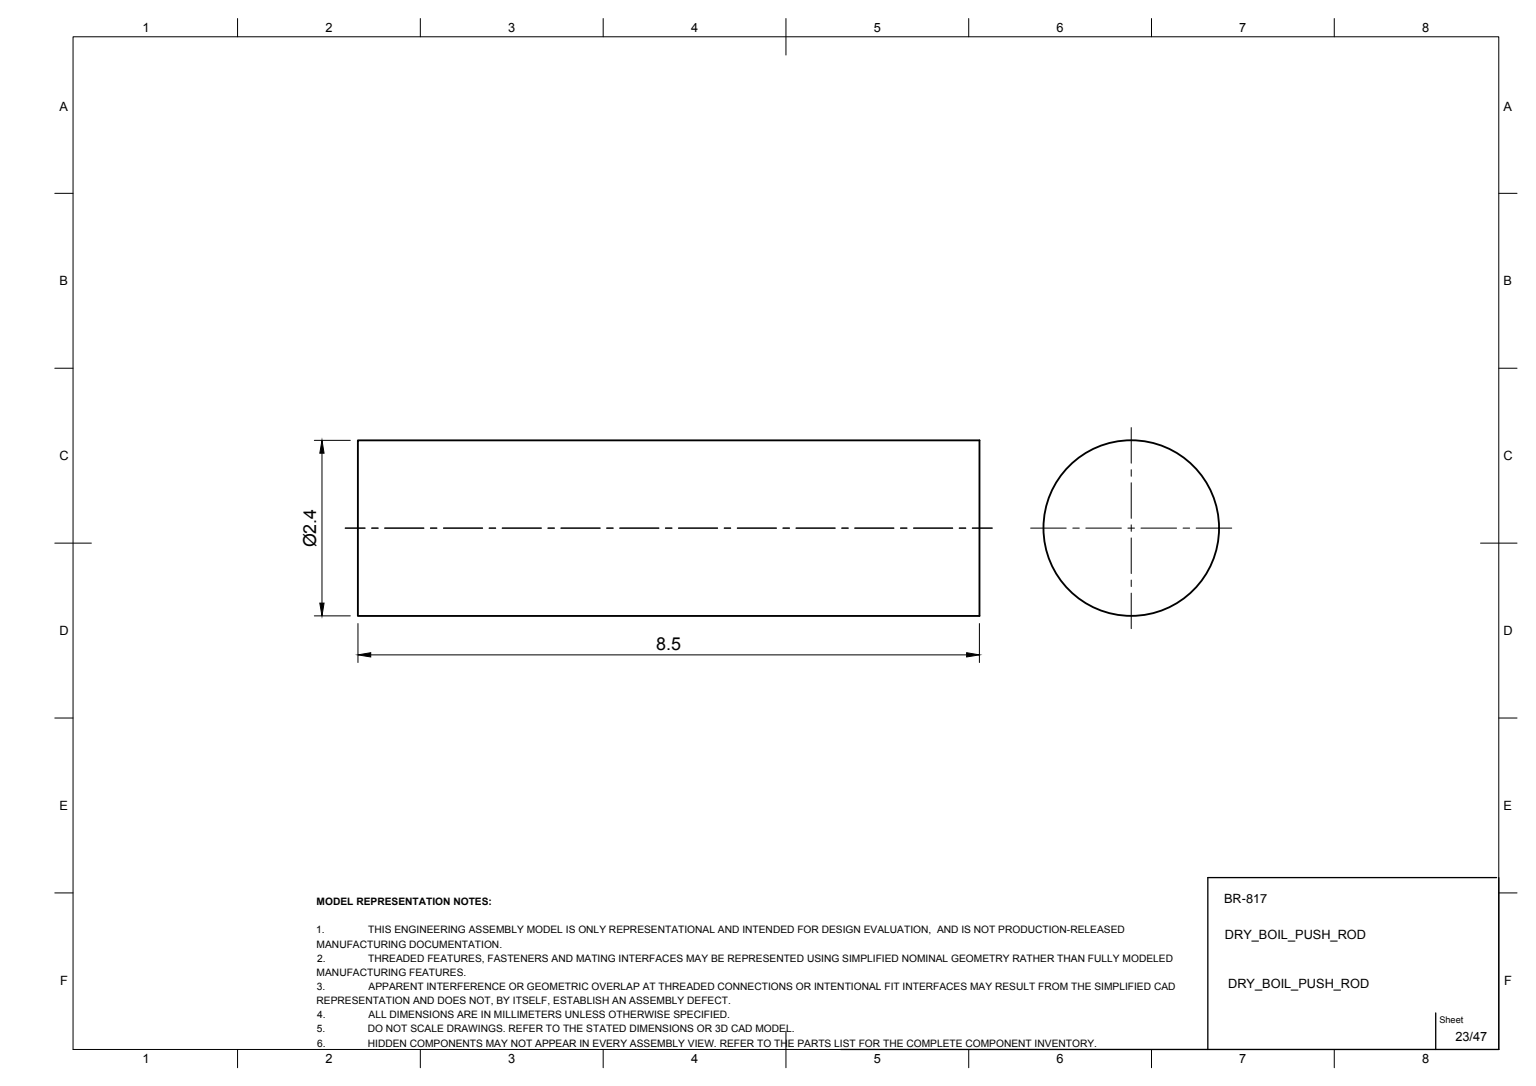
ISO-10303-21;
HEADER;
FILE_DESCRIPTION((''),'2;1');
FILE_NAME('DRY_BOIL_PUSH_ROD.step','2026-10-01T22:07:29-07:00',(''),(''),'','','');
FILE_SCHEMA (('AUTOMOTIVE_DESIGN { 1 0 10303 214 3 1 1 }'));
ENDSEC;
DATA;
#10=MECHANICAL_DESIGN_GEOMETRIC_PRESENTATION_REPRESENTATION('',(#557),#15484);
#487=SHAPE_REPRESENTATION_RELATIONSHIP('SRR','None',#15636,#522) ;
#522=ADVANCED_BREP_SHAPE_REPRESENTATION('',(#598),#15460) ;
#557=STYLED_ITEM('',(#15832),#598) ;
#598=MANIFOLD_SOLID_BREP('DRY_BOIL_PUSH_ROD',#8268) ;
#681=CYLINDRICAL_SURFACE('',#8996,0.12) ;
#1005=CIRCLE('',#8997,0.12) ;
#1006=CIRCLE('',#8998,0.12) ;
#1532=FACE_OUTER_BOUND('',#2088,.T.) ;
#1533=FACE_OUTER_BOUND('',#2089,.T.) ;
#1534=FACE_OUTER_BOUND('',#2090,.T.) ;
#2088=EDGE_LOOP('',(#5937,#5938,#5939,#5940)) ;
#2089=EDGE_LOOP('',(#5941)) ;
#2090=EDGE_LOOP('',(#5942)) ;
#2648=LINE('',#13678,#3122) ;
#3122=VECTOR('',#10765,0.12) ;
#3611=VERTEX_POINT('',#13675) ;
#3612=VERTEX_POINT('',#13677) ;
#4473=EDGE_CURVE('',#3611,#3611,#1005,.T.) ;
#4474=EDGE_CURVE('',#3611,#3612,#2648,.T.) ;
#4475=EDGE_CURVE('',#3612,#3612,#1006,.T.) ;
#5937=ORIENTED_EDGE('',*,*,#4473,.F.) ;
#5938=ORIENTED_EDGE('',*,*,#4474,.T.) ;
#5939=ORIENTED_EDGE('',*,*,#4475,.F.) ;
#5940=ORIENTED_EDGE('',*,*,#4474,.F.) ;
#5941=ORIENTED_EDGE('',*,*,#4475,.T.) ;
#5942=ORIENTED_EDGE('',*,*,#4473,.T.) ;
#7643=PLANE('',#8999) ;
#7644=PLANE('',#9000) ;
#7919=ADVANCED_FACE('',(#1532),#681,.T.) ;
#7920=ADVANCED_FACE('',(#1533),#7643,.T.) ;
#7921=ADVANCED_FACE('',(#1534),#7644,.T.) ;
#8268=CLOSED_SHELL('',(#7919,#7920,#7921)) ;
#8995=AXIS2_PLACEMENT_3D('',#13673,#10759,#10760) ;
#8996=AXIS2_PLACEMENT_3D('',#13674,#10761,#10762) ;
#8997=AXIS2_PLACEMENT_3D('',#13676,#10763,#10764) ;
#8998=AXIS2_PLACEMENT_3D('',#13679,#10766,#10767) ;
#8999=AXIS2_PLACEMENT_3D('',#13680,#10768,#10769) ;
#9000=AXIS2_PLACEMENT_3D('',#13681,#10770,#10771) ;
#10759=DIRECTION('axis',(0.,0.,1.)) ;
#10760=DIRECTION('refdir',(1.,0.,0.)) ;
#10761=DIRECTION('center_axis',(0.,0.,1.)) ;
#10762=DIRECTION('ref_axis',(1.,0.,0.)) ;
#10763=DIRECTION('center_axis',(0.,0.,1.)) ;
#10764=DIRECTION('ref_axis',(1.,0.,0.)) ;
#10765=DIRECTION('',(0.,0.,-1.)) ;
#10766=DIRECTION('center_axis',(0.,0.,-1.)) ;
#10767=DIRECTION('ref_axis',(1.,0.,0.)) ;
#10768=DIRECTION('center_axis',(0.,0.,-1.)) ;
#10769=DIRECTION('ref_axis',(-1.,0.,0.)) ;
#10770=DIRECTION('center_axis',(0.,0.,1.)) ;
#10771=DIRECTION('ref_axis',(1.,0.,0.)) ;
#13673=CARTESIAN_POINT('',(0.,0.,0.)) ;
#13674=CARTESIAN_POINT('Origin',(0.,-1.4,0.825)) ;
#13675=CARTESIAN_POINT('',(-0.12,-1.4,1.25)) ;
#13676=CARTESIAN_POINT('Origin',(0.,-1.4,1.25)) ;
#13677=CARTESIAN_POINT('',(-0.12,-1.4,0.4)) ;
#13678=CARTESIAN_POINT('',(-0.12,-1.4,0.825)) ;
#13679=CARTESIAN_POINT('Origin',(0.,-1.4,0.4)) ;
#13680=CARTESIAN_POINT('Origin',(0.,-1.4,0.4)) ;
#13681=CARTESIAN_POINT('Origin',(0.,-1.4,1.25)) ;
#15417=UNCERTAINTY_MEASURE_WITH_UNIT(LENGTH_MEASURE(0.001),#15485,
'DISTANCE_ACCURACY_VALUE',
'Maximum model space distance between geometric entities at asserted c
onnectivities') ;
#15441=UNCERTAINTY_MEASURE_WITH_UNIT(LENGTH_MEASURE(0.001),#15485,
'DISTANCE_ACCURACY_VALUE',
'Maximum model space distance between geometric entities at asserted c
onnectivities') ;
#15460=(
GEOMETRIC_REPRESENTATION_CONTEXT(3)
GLOBAL_UNCERTAINTY_ASSIGNED_CONTEXT((#15417))
GLOBAL_UNIT_ASSIGNED_CONTEXT((#15485,#15487,#15488))
REPRESENTATION_CONTEXT('','3D')
) ;
#15484=(
GEOMETRIC_REPRESENTATION_CONTEXT(3)
GLOBAL_UNCERTAINTY_ASSIGNED_CONTEXT((#15441))
GLOBAL_UNIT_ASSIGNED_CONTEXT((#15485,#15487,#15488))
REPRESENTATION_CONTEXT('','3D')
) ;
#15485=(
LENGTH_UNIT()
NAMED_UNIT(*)
SI_UNIT(.CENTI.,.METRE.)
) ;
#15487=(
NAMED_UNIT(*)
PLANE_ANGLE_UNIT()
SI_UNIT($,.RADIAN.)
) ;
#15488=(
NAMED_UNIT(*)
SI_UNIT($,.STERADIAN.)
SOLID_ANGLE_UNIT()
) ;
#15507=SHAPE_DEFINITION_REPRESENTATION(#15555,#15636) ;
#15555=PRODUCT_DEFINITION_SHAPE('',$,#15679) ;
#15636=SHAPE_REPRESENTATION('',(#8995),#15460) ;
#15660=PRODUCT_DEFINITION_CONTEXT('part definition',#15788,'design') ;
#15679=PRODUCT_DEFINITION('DRY_BOIL_PUSH_ROD','DRY_BOIL_PUSH_ROD',
#15721,#15660) ;
#15721=PRODUCT_DEFINITION_FORMATION('',$,#15808) ;
#15788=APPLICATION_CONTEXT(
'Core Data for Automotive Mechanical Design Process') ;
#15789=PRODUCT_CONTEXT('part definition',#15788,'mechanical') ;
#15808=PRODUCT('DRY_BOIL_PUSH_ROD','DRY_BOIL_PUSH_ROD',$,(#15789)) ;
#15832=PRESENTATION_STYLE_ASSIGNMENT((#15844)) ;
#15844=SURFACE_STYLE_USAGE(.BOTH.,#15856) ;
#15856=SURFACE_SIDE_STYLE('',(#15868)) ;
#15868=SURFACE_STYLE_FILL_AREA(#15880) ;
#15880=FILL_AREA_STYLE('Steel - Satin',(#15892)) ;
#15892=FILL_AREA_STYLE_COLOUR('Steel - Satin',#15904) ;
#15904=COLOUR_RGB('Steel - Satin', 0.72549020, 0.75294118, 0.79215686) ;
ENDSEC;
END-ISO-10303-21;
